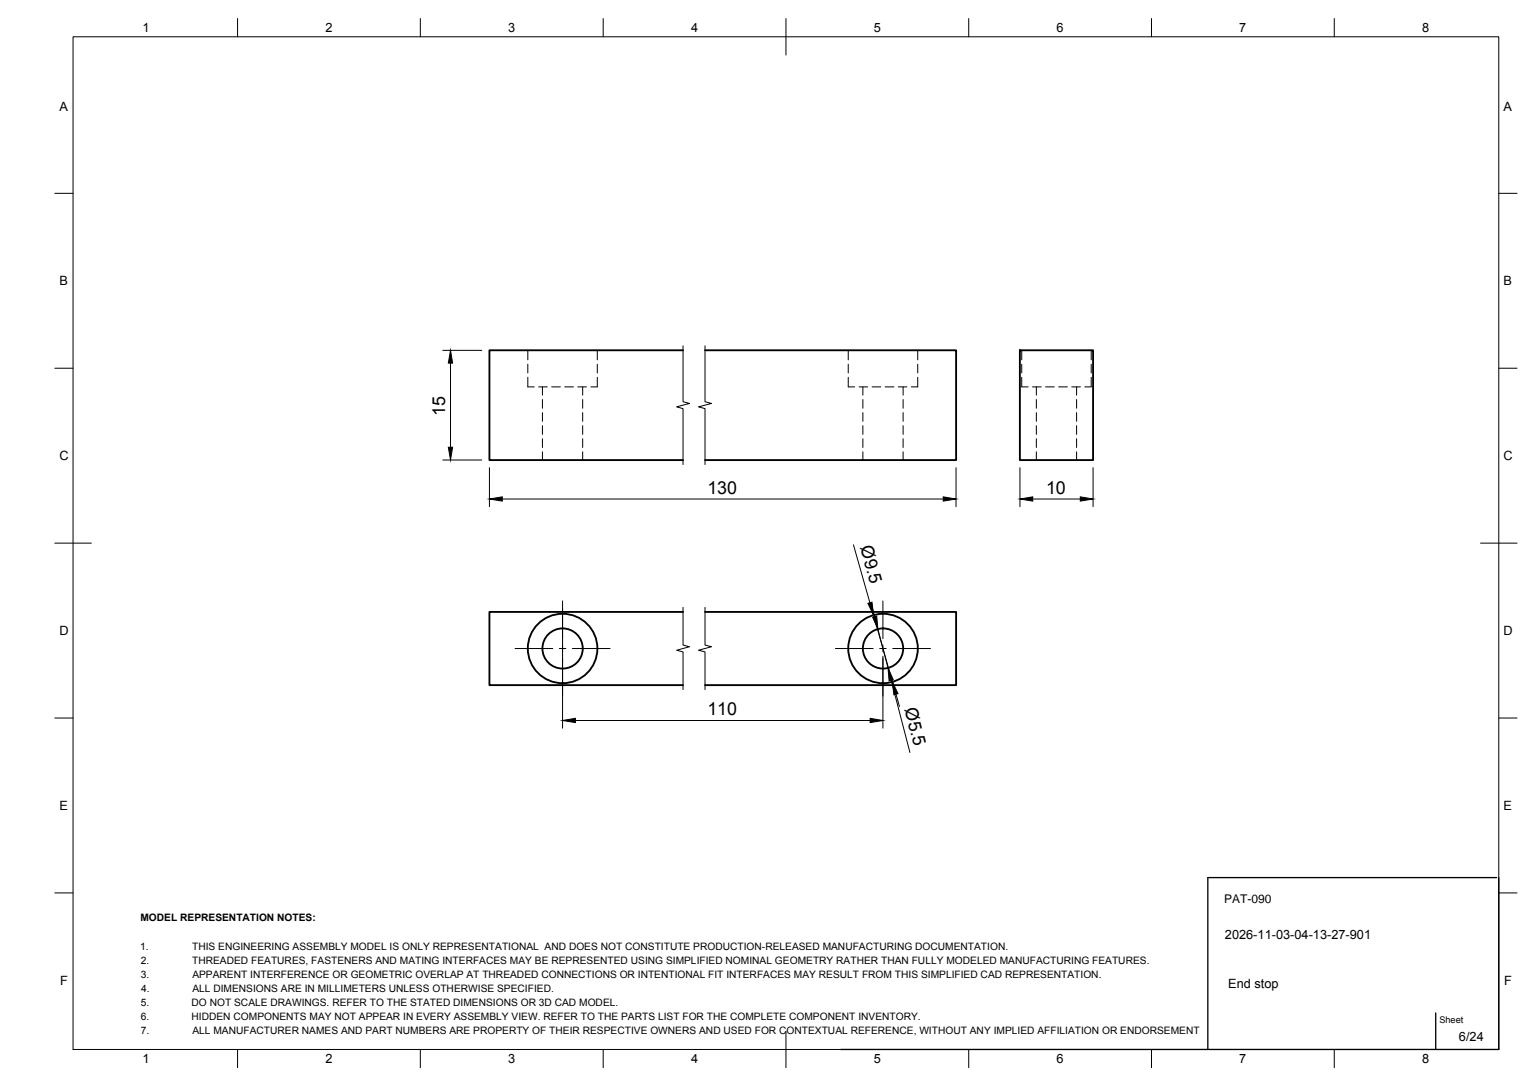
ISO-10303-21;
HEADER;
/* Generated by software containing ST-Developer
 * from STEP Tools, Inc. (www.steptools.com) 
 */

FILE_DESCRIPTION(
/* description */ ('Round-Shaft Linear Stage with Ball Bushings'),
/* implementation_level */ '2;1');

FILE_NAME(
/* name */ 'End stop.step',
/* time_stamp */ '2026-10-27T10:47:55-07:00',
/* author */ (''),
/* organization */ (''),
/* preprocessor_version */ 'ST-DEVELOPER v20.2',
/* originating_system */ 'Autodesk Translation Framework v15.17.0.0',
/* authorisation */ '');

FILE_SCHEMA (('AUTOMOTIVE_DESIGN { 1 0 10303 214 3 1 1 }'));
ENDSEC;

DATA;
#10=MECHANICAL_DESIGN_GEOMETRIC_PRESENTATION_REPRESENTATION('',(#303),#7835);
#261=SHAPE_REPRESENTATION_RELATIONSHIP('SRR','None',#7949,#282);
#282=ADVANCED_BREP_SHAPE_REPRESENTATION('',(#324),#7813);
#303=STYLED_ITEM('',(#8137),#324);
#324=MANIFOLD_SOLID_BREP('Body1',#4393);
#364=FACE_BOUND('',#917,.T.);
#365=FACE_BOUND('',#920,.T.);
#366=FACE_BOUND('',#928,.T.);
#367=FACE_BOUND('',#929,.T.);
#368=FACE_BOUND('',#931,.T.);
#369=FACE_BOUND('',#932,.T.);
#465=PLANE('',#4698);
#466=PLANE('',#4703);
#467=PLANE('',#4709);
#468=PLANE('',#4710);
#469=PLANE('',#4711);
#470=PLANE('',#4712);
#471=PLANE('',#4713);
#472=PLANE('',#4714);
#634=FACE_OUTER_BOUND('',#915,.T.);
#635=FACE_OUTER_BOUND('',#916,.T.);
#636=FACE_OUTER_BOUND('',#918,.T.);
#637=FACE_OUTER_BOUND('',#919,.T.);
#638=FACE_OUTER_BOUND('',#921,.T.);
#639=FACE_OUTER_BOUND('',#922,.T.);
#640=FACE_OUTER_BOUND('',#923,.T.);
#641=FACE_OUTER_BOUND('',#924,.T.);
#642=FACE_OUTER_BOUND('',#925,.T.);
#643=FACE_OUTER_BOUND('',#926,.T.);
#644=FACE_OUTER_BOUND('',#927,.T.);
#645=FACE_OUTER_BOUND('',#930,.T.);
#915=EDGE_LOOP('',(#3090,#3091,#3092,#3093));
#916=EDGE_LOOP('',(#3094));
#917=EDGE_LOOP('',(#3095));
#918=EDGE_LOOP('',(#3096,#3097,#3098,#3099));
#919=EDGE_LOOP('',(#3100));
#920=EDGE_LOOP('',(#3101));
#921=EDGE_LOOP('',(#3102,#3103,#3104,#3105));
#922=EDGE_LOOP('',(#3106,#3107,#3108,#3109));
#923=EDGE_LOOP('',(#3110,#3111,#3112,#3113));
#924=EDGE_LOOP('',(#3114,#3115,#3116,#3117));
#925=EDGE_LOOP('',(#3118,#3119,#3120,#3121));
#926=EDGE_LOOP('',(#3122,#3123,#3124,#3125));
#927=EDGE_LOOP('',(#3126,#3127,#3128,#3129));
#928=EDGE_LOOP('',(#3130));
#929=EDGE_LOOP('',(#3131));
#930=EDGE_LOOP('',(#3132,#3133,#3134,#3135));
#931=EDGE_LOOP('',(#3136));
#932=EDGE_LOOP('',(#3137));
#1273=LINE('',#6676,#1613);
#1274=LINE('',#6685,#1614);
#1275=LINE('',#6693,#1615);
#1276=LINE('',#6697,#1616);
#1277=LINE('',#6701,#1617);
#1278=LINE('',#6703,#1618);
#1279=LINE('',#6705,#1619);
#1280=LINE('',#6706,#1620);
#1281=LINE('',#6709,#1621);
#1282=LINE('',#6711,#1622);
#1283=LINE('',#6712,#1623);
#1284=LINE('',#6715,#1624);
#1285=LINE('',#6717,#1625);
#1286=LINE('',#6718,#1626);
#1287=LINE('',#6720,#1627);
#1288=LINE('',#6721,#1628);
#1613=VECTOR('',#5296,0.475);
#1614=VECTOR('',#5307,0.475);
#1615=VECTOR('',#5318,0.275);
#1616=VECTOR('',#5323,0.275);
#1617=VECTOR('',#5326,1.);
#1618=VECTOR('',#5327,1.);
#1619=VECTOR('',#5328,1.);
#1620=VECTOR('',#5329,1.);
#1621=VECTOR('',#5332,1.);
#1622=VECTOR('',#5333,1.);
#1623=VECTOR('',#5334,1.);
#1624=VECTOR('',#5337,1.);
#1625=VECTOR('',#5338,1.);
#1626=VECTOR('',#5339,1.);
#1627=VECTOR('',#5342,1.);
#1628=VECTOR('',#5343,1.);
#1953=CIRCLE('',#4696,0.475);
#1954=CIRCLE('',#4697,0.475);
#1955=CIRCLE('',#4699,0.275);
#1956=CIRCLE('',#4701,0.475);
#1957=CIRCLE('',#4702,0.475);
#1958=CIRCLE('',#4704,0.275);
#1959=CIRCLE('',#4706,0.275);
#1960=CIRCLE('',#4708,0.275);
#2150=VERTEX_POINT('',#6673);
#2151=VERTEX_POINT('',#6675);
#2152=VERTEX_POINT('',#6679);
#2153=VERTEX_POINT('',#6682);
#2154=VERTEX_POINT('',#6684);
#2155=VERTEX_POINT('',#6688);
#2156=VERTEX_POINT('',#6691);
#2157=VERTEX_POINT('',#6695);
#2158=VERTEX_POINT('',#6699);
#2159=VERTEX_POINT('',#6700);
#2160=VERTEX_POINT('',#6702);
#2161=VERTEX_POINT('',#6704);
#2162=VERTEX_POINT('',#6708);
#2163=VERTEX_POINT('',#6710);
#2164=VERTEX_POINT('',#6714);
#2165=VERTEX_POINT('',#6716);
#2513=EDGE_CURVE('',#2150,#2150,#1953,.T.);
#2514=EDGE_CURVE('',#2150,#2151,#1273,.T.);
#2515=EDGE_CURVE('',#2151,#2151,#1954,.T.);
#2516=EDGE_CURVE('',#2152,#2152,#1955,.T.);
#2517=EDGE_CURVE('',#2153,#2153,#1956,.T.);
#2518=EDGE_CURVE('',#2153,#2154,#1274,.T.);
#2519=EDGE_CURVE('',#2154,#2154,#1957,.T.);
#2520=EDGE_CURVE('',#2155,#2155,#1958,.T.);
#2521=EDGE_CURVE('',#2156,#2156,#1959,.T.);
#2522=EDGE_CURVE('',#2156,#2152,#1275,.T.);
#2523=EDGE_CURVE('',#2157,#2157,#1960,.T.);
#2524=EDGE_CURVE('',#2157,#2155,#1276,.T.);
#2525=EDGE_CURVE('',#2158,#2159,#1277,.T.);
#2526=EDGE_CURVE('',#2159,#2160,#1278,.T.);
#2527=EDGE_CURVE('',#2161,#2160,#1279,.T.);
#2528=EDGE_CURVE('',#2158,#2161,#1280,.T.);
#2529=EDGE_CURVE('',#2162,#2158,#1281,.T.);
#2530=EDGE_CURVE('',#2163,#2161,#1282,.T.);
#2531=EDGE_CURVE('',#2162,#2163,#1283,.T.);
#2532=EDGE_CURVE('',#2164,#2162,#1284,.T.);
#2533=EDGE_CURVE('',#2165,#2163,#1285,.T.);
#2534=EDGE_CURVE('',#2164,#2165,#1286,.T.);
#2535=EDGE_CURVE('',#2159,#2164,#1287,.T.);
#2536=EDGE_CURVE('',#2160,#2165,#1288,.T.);
#3090=ORIENTED_EDGE('',*,*,#2513,.F.);
#3091=ORIENTED_EDGE('',*,*,#2514,.T.);
#3092=ORIENTED_EDGE('',*,*,#2515,.F.);
#3093=ORIENTED_EDGE('',*,*,#2514,.F.);
#3094=ORIENTED_EDGE('',*,*,#2513,.T.);
#3095=ORIENTED_EDGE('',*,*,#2516,.F.);
#3096=ORIENTED_EDGE('',*,*,#2517,.F.);
#3097=ORIENTED_EDGE('',*,*,#2518,.T.);
#3098=ORIENTED_EDGE('',*,*,#2519,.F.);
#3099=ORIENTED_EDGE('',*,*,#2518,.F.);
#3100=ORIENTED_EDGE('',*,*,#2517,.T.);
#3101=ORIENTED_EDGE('',*,*,#2520,.F.);
#3102=ORIENTED_EDGE('',*,*,#2521,.F.);
#3103=ORIENTED_EDGE('',*,*,#2522,.T.);
#3104=ORIENTED_EDGE('',*,*,#2516,.T.);
#3105=ORIENTED_EDGE('',*,*,#2522,.F.);
#3106=ORIENTED_EDGE('',*,*,#2523,.F.);
#3107=ORIENTED_EDGE('',*,*,#2524,.T.);
#3108=ORIENTED_EDGE('',*,*,#2520,.T.);
#3109=ORIENTED_EDGE('',*,*,#2524,.F.);
#3110=ORIENTED_EDGE('',*,*,#2525,.T.);
#3111=ORIENTED_EDGE('',*,*,#2526,.T.);
#3112=ORIENTED_EDGE('',*,*,#2527,.F.);
#3113=ORIENTED_EDGE('',*,*,#2528,.F.);
#3114=ORIENTED_EDGE('',*,*,#2529,.T.);
#3115=ORIENTED_EDGE('',*,*,#2528,.T.);
#3116=ORIENTED_EDGE('',*,*,#2530,.F.);
#3117=ORIENTED_EDGE('',*,*,#2531,.F.);
#3118=ORIENTED_EDGE('',*,*,#2532,.T.);
#3119=ORIENTED_EDGE('',*,*,#2531,.T.);
#3120=ORIENTED_EDGE('',*,*,#2533,.F.);
#3121=ORIENTED_EDGE('',*,*,#2534,.F.);
#3122=ORIENTED_EDGE('',*,*,#2535,.T.);
#3123=ORIENTED_EDGE('',*,*,#2534,.T.);
#3124=ORIENTED_EDGE('',*,*,#2536,.F.);
#3125=ORIENTED_EDGE('',*,*,#2526,.F.);
#3126=ORIENTED_EDGE('',*,*,#2536,.T.);
#3127=ORIENTED_EDGE('',*,*,#2533,.T.);
#3128=ORIENTED_EDGE('',*,*,#2530,.T.);
#3129=ORIENTED_EDGE('',*,*,#2527,.T.);
#3130=ORIENTED_EDGE('',*,*,#2515,.T.);
#3131=ORIENTED_EDGE('',*,*,#2519,.T.);
#3132=ORIENTED_EDGE('',*,*,#2535,.F.);
#3133=ORIENTED_EDGE('',*,*,#2525,.F.);
#3134=ORIENTED_EDGE('',*,*,#2529,.F.);
#3135=ORIENTED_EDGE('',*,*,#2532,.F.);
#3136=ORIENTED_EDGE('',*,*,#2521,.T.);
#3137=ORIENTED_EDGE('',*,*,#2523,.T.);
#4064=CYLINDRICAL_SURFACE('',#4695,0.475);
#4065=CYLINDRICAL_SURFACE('',#4700,0.475);
#4066=CYLINDRICAL_SURFACE('',#4705,0.275);
#4067=CYLINDRICAL_SURFACE('',#4707,0.275);
#4153=ADVANCED_FACE('',(#634),#4064,.F.);
#4154=ADVANCED_FACE('',(#635,#364),#465,.T.);
#4155=ADVANCED_FACE('',(#636),#4065,.F.);
#4156=ADVANCED_FACE('',(#637,#365),#466,.T.);
#4157=ADVANCED_FACE('',(#638),#4066,.F.);
#4158=ADVANCED_FACE('',(#639),#4067,.F.);
#4159=ADVANCED_FACE('',(#640),#467,.T.);
#4160=ADVANCED_FACE('',(#641),#468,.T.);
#4161=ADVANCED_FACE('',(#642),#469,.T.);
#4162=ADVANCED_FACE('',(#643),#470,.T.);
#4163=ADVANCED_FACE('',(#644,#366,#367),#471,.T.);
#4164=ADVANCED_FACE('',(#645,#368,#369),#472,.F.);
#4393=CLOSED_SHELL('',(#4153,#4154,#4155,#4156,#4157,#4158,#4159,#4160,
#4161,#4162,#4163,#4164));
#4694=AXIS2_PLACEMENT_3D('',#6671,#5290,#5291);
#4695=AXIS2_PLACEMENT_3D('',#6672,#5292,#5293);
#4696=AXIS2_PLACEMENT_3D('',#6674,#5294,#5295);
#4697=AXIS2_PLACEMENT_3D('',#6677,#5297,#5298);
#4698=AXIS2_PLACEMENT_3D('',#6678,#5299,#5300);
#4699=AXIS2_PLACEMENT_3D('',#6680,#5301,#5302);
#4700=AXIS2_PLACEMENT_3D('',#6681,#5303,#5304);
#4701=AXIS2_PLACEMENT_3D('',#6683,#5305,#5306);
#4702=AXIS2_PLACEMENT_3D('',#6686,#5308,#5309);
#4703=AXIS2_PLACEMENT_3D('',#6687,#5310,#5311);
#4704=AXIS2_PLACEMENT_3D('',#6689,#5312,#5313);
#4705=AXIS2_PLACEMENT_3D('',#6690,#5314,#5315);
#4706=AXIS2_PLACEMENT_3D('',#6692,#5316,#5317);
#4707=AXIS2_PLACEMENT_3D('',#6694,#5319,#5320);
#4708=AXIS2_PLACEMENT_3D('',#6696,#5321,#5322);
#4709=AXIS2_PLACEMENT_3D('',#6698,#5324,#5325);
#4710=AXIS2_PLACEMENT_3D('',#6707,#5330,#5331);
#4711=AXIS2_PLACEMENT_3D('',#6713,#5335,#5336);
#4712=AXIS2_PLACEMENT_3D('',#6719,#5340,#5341);
#4713=AXIS2_PLACEMENT_3D('',#6722,#5344,#5345);
#4714=AXIS2_PLACEMENT_3D('',#6723,#5346,#5347);
#5290=DIRECTION('axis',(0.,0.,1.));
#5291=DIRECTION('refdir',(1.,0.,0.));
#5292=DIRECTION('center_axis',(0.,0.,1.));
#5293=DIRECTION('ref_axis',(1.,0.,0.));
#5294=DIRECTION('center_axis',(0.,0.,1.));
#5295=DIRECTION('ref_axis',(1.,0.,0.));
#5296=DIRECTION('',(0.,0.,1.));
#5297=DIRECTION('center_axis',(0.,0.,-1.));
#5298=DIRECTION('ref_axis',(1.,0.,0.));
#5299=DIRECTION('center_axis',(0.,0.,1.));
#5300=DIRECTION('ref_axis',(1.,0.,0.));
#5301=DIRECTION('center_axis',(0.,0.,1.));
#5302=DIRECTION('ref_axis',(1.,0.,0.));
#5303=DIRECTION('center_axis',(0.,0.,1.));
#5304=DIRECTION('ref_axis',(1.,0.,0.));
#5305=DIRECTION('center_axis',(0.,0.,1.));
#5306=DIRECTION('ref_axis',(1.,0.,0.));
#5307=DIRECTION('',(0.,0.,1.));
#5308=DIRECTION('center_axis',(0.,0.,-1.));
#5309=DIRECTION('ref_axis',(1.,0.,0.));
#5310=DIRECTION('center_axis',(0.,0.,1.));
#5311=DIRECTION('ref_axis',(1.,0.,0.));
#5312=DIRECTION('center_axis',(0.,0.,1.));
#5313=DIRECTION('ref_axis',(1.,0.,0.));
#5314=DIRECTION('center_axis',(0.,0.,1.));
#5315=DIRECTION('ref_axis',(1.,0.,0.));
#5316=DIRECTION('center_axis',(0.,0.,1.));
#5317=DIRECTION('ref_axis',(1.,0.,0.));
#5318=DIRECTION('',(0.,0.,1.));
#5319=DIRECTION('center_axis',(0.,0.,1.));
#5320=DIRECTION('ref_axis',(1.,0.,0.));
#5321=DIRECTION('center_axis',(0.,0.,1.));
#5322=DIRECTION('ref_axis',(1.,0.,0.));
#5323=DIRECTION('',(0.,0.,1.));
#5324=DIRECTION('center_axis',(0.,1.,0.));
#5325=DIRECTION('ref_axis',(-1.,0.,0.));
#5326=DIRECTION('',(-1.,0.,0.));
#5327=DIRECTION('',(0.,0.,1.));
#5328=DIRECTION('',(-1.,0.,0.));
#5329=DIRECTION('',(0.,0.,1.));
#5330=DIRECTION('center_axis',(1.,0.,0.));
#5331=DIRECTION('ref_axis',(0.,1.,0.));
#5332=DIRECTION('',(0.,1.,0.));
#5333=DIRECTION('',(0.,1.,0.));
#5334=DIRECTION('',(0.,0.,1.));
#5335=DIRECTION('center_axis',(0.,-1.,0.));
#5336=DIRECTION('ref_axis',(1.,0.,0.));
#5337=DIRECTION('',(1.,0.,0.));
#5338=DIRECTION('',(1.,0.,0.));
#5339=DIRECTION('',(0.,0.,1.));
#5340=DIRECTION('center_axis',(-1.,0.,0.));
#5341=DIRECTION('ref_axis',(0.,-1.,0.));
#5342=DIRECTION('',(0.,-1.,0.));
#5343=DIRECTION('',(0.,-1.,0.));
#5344=DIRECTION('center_axis',(0.,0.,1.));
#5345=DIRECTION('ref_axis',(1.,0.,0.));
#5346=DIRECTION('center_axis',(0.,0.,1.));
#5347=DIRECTION('ref_axis',(1.,0.,0.));
#6671=CARTESIAN_POINT('',(0.,0.,0.));
#6672=CARTESIAN_POINT('Origin',(3.5,-5.5,2.));
#6673=CARTESIAN_POINT('',(3.025,-5.5,2.));
#6674=CARTESIAN_POINT('Origin',(3.5,-5.5,2.));
#6675=CARTESIAN_POINT('',(3.025,-5.5,2.5));
#6676=CARTESIAN_POINT('',(3.025,-5.5,2.));
#6677=CARTESIAN_POINT('Origin',(3.5,-5.5,2.5));
#6678=CARTESIAN_POINT('Origin',(3.5,-5.5,2.));
#6679=CARTESIAN_POINT('',(3.225,-5.5,2.));
#6680=CARTESIAN_POINT('Origin',(3.5,-5.5,2.));
#6681=CARTESIAN_POINT('Origin',(3.5,5.5,2.));
#6682=CARTESIAN_POINT('',(3.025,5.5,2.));
#6683=CARTESIAN_POINT('Origin',(3.5,5.5,2.));
#6684=CARTESIAN_POINT('',(3.025,5.5,2.5));
#6685=CARTESIAN_POINT('',(3.025,5.5,2.));
#6686=CARTESIAN_POINT('Origin',(3.5,5.5,2.5));
#6687=CARTESIAN_POINT('Origin',(3.5,5.5,2.));
#6688=CARTESIAN_POINT('',(3.225,5.5,2.));
#6689=CARTESIAN_POINT('Origin',(3.5,5.5,2.));
#6690=CARTESIAN_POINT('Origin',(3.5,-5.5,0.9));
#6691=CARTESIAN_POINT('',(3.225,-5.5,1.));
#6692=CARTESIAN_POINT('Origin',(3.5,-5.5,1.));
#6693=CARTESIAN_POINT('',(3.225,-5.5,0.9));
#6694=CARTESIAN_POINT('Origin',(3.5,5.5,0.9));
#6695=CARTESIAN_POINT('',(3.225,5.5,1.));
#6696=CARTESIAN_POINT('Origin',(3.5,5.5,1.));
#6697=CARTESIAN_POINT('',(3.225,5.5,0.9));
#6698=CARTESIAN_POINT('Origin',(4.,6.5,1.));
#6699=CARTESIAN_POINT('',(4.,6.5,1.));
#6700=CARTESIAN_POINT('',(3.,6.5,1.));
#6701=CARTESIAN_POINT('',(4.,6.5,1.));
#6702=CARTESIAN_POINT('',(3.,6.5,2.5));
#6703=CARTESIAN_POINT('',(3.,6.5,1.));
#6704=CARTESIAN_POINT('',(4.,6.5,2.5));
#6705=CARTESIAN_POINT('',(4.,6.5,2.5));
#6706=CARTESIAN_POINT('',(4.,6.5,1.));
#6707=CARTESIAN_POINT('Origin',(4.,-6.5,1.));
#6708=CARTESIAN_POINT('',(4.,-6.5,1.));
#6709=CARTESIAN_POINT('',(4.,-6.5,1.));
#6710=CARTESIAN_POINT('',(4.,-6.5,2.5));
#6711=CARTESIAN_POINT('',(4.,-6.5,2.5));
#6712=CARTESIAN_POINT('',(4.,-6.5,1.));
#6713=CARTESIAN_POINT('Origin',(3.,-6.5,1.));
#6714=CARTESIAN_POINT('',(3.,-6.5,1.));
#6715=CARTESIAN_POINT('',(3.,-6.5,1.));
#6716=CARTESIAN_POINT('',(3.,-6.5,2.5));
#6717=CARTESIAN_POINT('',(3.,-6.5,2.5));
#6718=CARTESIAN_POINT('',(3.,-6.5,1.));
#6719=CARTESIAN_POINT('Origin',(3.,6.5,1.));
#6720=CARTESIAN_POINT('',(3.,6.5,1.));
#6721=CARTESIAN_POINT('',(3.,6.5,2.5));
#6722=CARTESIAN_POINT('Origin',(3.5,0.,2.5));
#6723=CARTESIAN_POINT('Origin',(3.5,0.,1.));
#7787=UNCERTAINTY_MEASURE_WITH_UNIT(LENGTH_MEASURE(0.001),#7836,
'DISTANCE_ACCURACY_VALUE',
'Maximum model space distance between geometric entities at asserted c
onnectivities');
#7809=UNCERTAINTY_MEASURE_WITH_UNIT(LENGTH_MEASURE(0.001),#7836,
'DISTANCE_ACCURACY_VALUE',
'Maximum model space distance between geometric entities at asserted c
onnectivities');
#7813=(
GEOMETRIC_REPRESENTATION_CONTEXT(3)
GLOBAL_UNCERTAINTY_ASSIGNED_CONTEXT((#7787))
GLOBAL_UNIT_ASSIGNED_CONTEXT((#7836,#7838,#7839))
REPRESENTATION_CONTEXT('','3D')
);
#7835=(
GEOMETRIC_REPRESENTATION_CONTEXT(3)
GLOBAL_UNCERTAINTY_ASSIGNED_CONTEXT((#7809))
GLOBAL_UNIT_ASSIGNED_CONTEXT((#7836,#7838,#7839))
REPRESENTATION_CONTEXT('','3D')
);
#7836=(
LENGTH_UNIT()
NAMED_UNIT(*)
SI_UNIT(.CENTI.,.METRE.)
);
#7838=(
NAMED_UNIT(*)
PLANE_ANGLE_UNIT()
SI_UNIT($,.RADIAN.)
);
#7839=(
NAMED_UNIT(*)
SI_UNIT($,.STERADIAN.)
SOLID_ANGLE_UNIT()
);
#7843=SHAPE_DEFINITION_REPRESENTATION(#7868,#7949);
#7868=PRODUCT_DEFINITION_SHAPE('',$,#7975);
#7949=SHAPE_REPRESENTATION('',(#4694),#7813);
#7971=PRODUCT_DEFINITION_CONTEXT('part definition',#8048,'design');
#7975=PRODUCT_DEFINITION('End stop','End stop',#8000,#7971);
#8000=PRODUCT_DEFINITION_FORMATION('',$,#8053);
#8048=APPLICATION_CONTEXT(
'Core Data for Automotive Mechanical Design Process');
#8049=PRODUCT_CONTEXT('part definition',#8048,'mechanical');
#8053=PRODUCT('End stop','End stop','End stop',(#8049));
#8131=COLOUR_RGB('Sky Blue',0.24,0.69,0.87);
#8132=FILL_AREA_STYLE_COLOUR('',#8131);
#8133=FILL_AREA_STYLE('',(#8132));
#8134=SURFACE_STYLE_FILL_AREA(#8133);
#8135=SURFACE_SIDE_STYLE('',(#8134));
#8136=SURFACE_STYLE_USAGE(.BOTH.,#8135);
#8137=PRESENTATION_STYLE_ASSIGNMENT((#8136));
ENDSEC;
END-ISO-10303-21;
